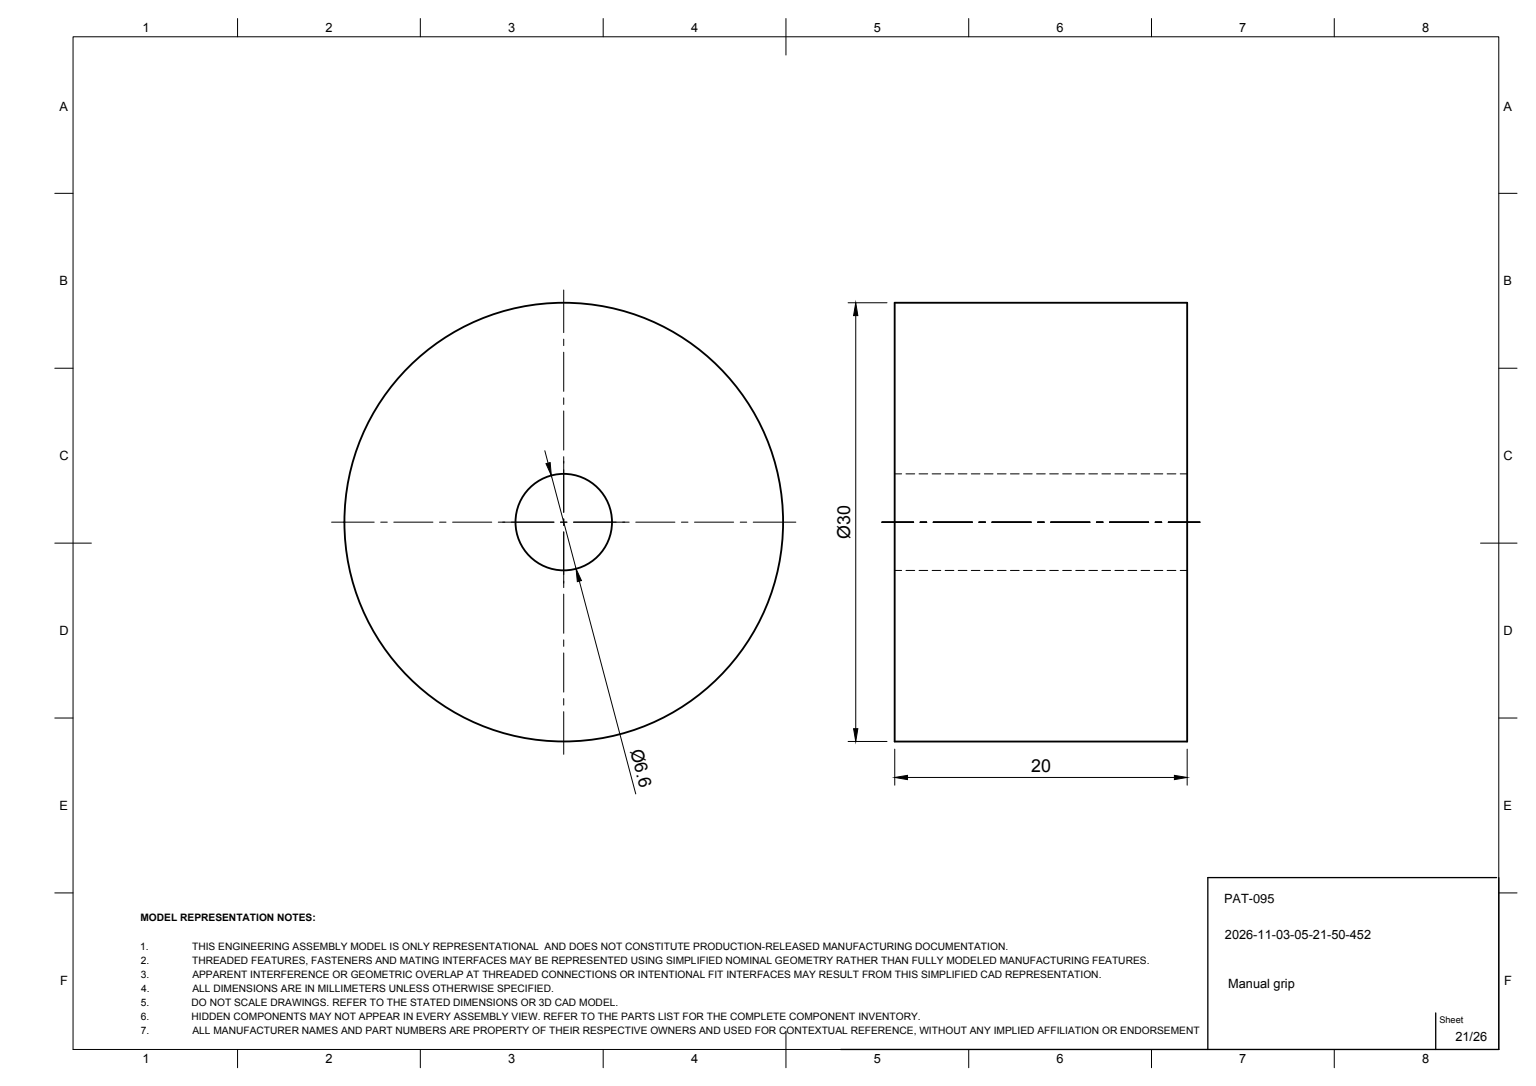
ISO-10303-21;
HEADER;
/* Generated by software containing ST-Developer
 * from STEP Tools, Inc. (www.steptools.com) 
 */

FILE_DESCRIPTION(
/* description */ ('Single-Axis Profile-Rail Linear Slide'),
/* implementation_level */ '2;1');

FILE_NAME(
/* name */ 'Manual grip.step',
/* time_stamp */ '2026-10-27T10:47:43-07:00',
/* author */ (''),
/* organization */ (''),
/* preprocessor_version */ 'ST-DEVELOPER v20.2',
/* originating_system */ 'Autodesk Translation Framework v15.17.0.0',
/* authorisation */ '');

FILE_SCHEMA (('AUTOMOTIVE_DESIGN { 1 0 10303 214 3 1 1 }'));
ENDSEC;

DATA;
#10=MECHANICAL_DESIGN_GEOMETRIC_PRESENTATION_REPRESENTATION('',(#346),#14478);
#292=SHAPE_REPRESENTATION_RELATIONSHIP('SRR','None',#14623,#319);
#319=ADVANCED_BREP_SHAPE_REPRESENTATION('',(#371),#14467);
#346=STYLED_ITEM('',(#14838),#371);
#371=MANIFOLD_SOLID_BREP('Body1',#8608);
#453=FACE_BOUND('',#1717,.T.);
#454=FACE_BOUND('',#1719,.T.);
#761=PLANE('',#9390);
#762=PLANE('',#9391);
#1184=FACE_OUTER_BOUND('',#1714,.T.);
#1185=FACE_OUTER_BOUND('',#1715,.T.);
#1186=FACE_OUTER_BOUND('',#1716,.T.);
#1187=FACE_OUTER_BOUND('',#1718,.T.);
#1714=EDGE_LOOP('',(#7583,#7584,#7585,#7586));
#1715=EDGE_LOOP('',(#7587,#7588,#7589,#7590));
#1716=EDGE_LOOP('',(#7591));
#1717=EDGE_LOOP('',(#7592));
#1718=EDGE_LOOP('',(#7593));
#1719=EDGE_LOOP('',(#7594));
#2625=LINE('',#13838,#3596);
#2626=LINE('',#13844,#3597);
#3596=VECTOR('',#11340,0.33);
#3597=VECTOR('',#11347,1.5);
#3880=CIRCLE('',#9385,0.33);
#3881=CIRCLE('',#9386,0.33);
#3882=CIRCLE('',#9388,1.5);
#3883=CIRCLE('',#9389,1.5);
#4526=VERTEX_POINT('',#13835);
#4527=VERTEX_POINT('',#13837);
#4528=VERTEX_POINT('',#13841);
#4529=VERTEX_POINT('',#13843);
#5569=EDGE_CURVE('',#4526,#4526,#3880,.T.);
#5570=EDGE_CURVE('',#4526,#4527,#2625,.T.);
#5571=EDGE_CURVE('',#4527,#4527,#3881,.T.);
#5572=EDGE_CURVE('',#4528,#4528,#3882,.T.);
#5573=EDGE_CURVE('',#4528,#4529,#2626,.T.);
#5574=EDGE_CURVE('',#4529,#4529,#3883,.T.);
#7583=ORIENTED_EDGE('',*,*,#5569,.F.);
#7584=ORIENTED_EDGE('',*,*,#5570,.T.);
#7585=ORIENTED_EDGE('',*,*,#5571,.T.);
#7586=ORIENTED_EDGE('',*,*,#5570,.F.);
#7587=ORIENTED_EDGE('',*,*,#5572,.F.);
#7588=ORIENTED_EDGE('',*,*,#5573,.T.);
#7589=ORIENTED_EDGE('',*,*,#5574,.T.);
#7590=ORIENTED_EDGE('',*,*,#5573,.F.);
#7591=ORIENTED_EDGE('',*,*,#5572,.T.);
#7592=ORIENTED_EDGE('',*,*,#5569,.T.);
#7593=ORIENTED_EDGE('',*,*,#5574,.F.);
#7594=ORIENTED_EDGE('',*,*,#5571,.F.);
#8116=CYLINDRICAL_SURFACE('',#9384,0.33);
#8117=CYLINDRICAL_SURFACE('',#9387,1.5);
#8478=ADVANCED_FACE('',(#1184),#8116,.F.);
#8479=ADVANCED_FACE('',(#1185),#8117,.T.);
#8480=ADVANCED_FACE('',(#1186,#453),#761,.T.);
#8481=ADVANCED_FACE('',(#1187,#454),#762,.F.);
#8608=CLOSED_SHELL('',(#8478,#8479,#8480,#8481));
#9383=AXIS2_PLACEMENT_3D('',#13833,#11334,#11335);
#9384=AXIS2_PLACEMENT_3D('',#13834,#11336,#11337);
#9385=AXIS2_PLACEMENT_3D('',#13836,#11338,#11339);
#9386=AXIS2_PLACEMENT_3D('',#13839,#11341,#11342);
#9387=AXIS2_PLACEMENT_3D('',#13840,#11343,#11344);
#9388=AXIS2_PLACEMENT_3D('',#13842,#11345,#11346);
#9389=AXIS2_PLACEMENT_3D('',#13845,#11348,#11349);
#9390=AXIS2_PLACEMENT_3D('',#13846,#11350,#11351);
#9391=AXIS2_PLACEMENT_3D('',#13847,#11352,#11353);
#11334=DIRECTION('axis',(0.,0.,1.));
#11335=DIRECTION('refdir',(1.,0.,0.));
#11336=DIRECTION('center_axis',(0.,0.,1.));
#11337=DIRECTION('ref_axis',(1.,0.,0.));
#11338=DIRECTION('center_axis',(0.,0.,-1.));
#11339=DIRECTION('ref_axis',(1.,0.,0.));
#11340=DIRECTION('',(0.,0.,-1.));
#11341=DIRECTION('center_axis',(0.,0.,-1.));
#11342=DIRECTION('ref_axis',(1.,0.,0.));
#11343=DIRECTION('center_axis',(0.,0.,1.));
#11344=DIRECTION('ref_axis',(1.,0.,0.));
#11345=DIRECTION('center_axis',(0.,0.,1.));
#11346=DIRECTION('ref_axis',(1.,0.,0.));
#11347=DIRECTION('',(0.,0.,-1.));
#11348=DIRECTION('center_axis',(0.,0.,1.));
#11349=DIRECTION('ref_axis',(1.,0.,0.));
#11350=DIRECTION('center_axis',(0.,0.,1.));
#11351=DIRECTION('ref_axis',(1.,0.,0.));
#11352=DIRECTION('center_axis',(0.,0.,1.));
#11353=DIRECTION('ref_axis',(1.,0.,0.));
#13833=CARTESIAN_POINT('',(0.,0.,0.));
#13834=CARTESIAN_POINT('Origin',(11.,0.,6.4));
#13835=CARTESIAN_POINT('',(10.67,-4.04133443718627E-17,8.4));
#13836=CARTESIAN_POINT('Origin',(11.,0.,8.4));
#13837=CARTESIAN_POINT('',(10.67,-4.04133443718627E-17,6.4));
#13838=CARTESIAN_POINT('',(10.67,-4.04133443718627E-17,6.4));
#13839=CARTESIAN_POINT('Origin',(11.,0.,6.4));
#13840=CARTESIAN_POINT('Origin',(11.,0.,6.4));
#13841=CARTESIAN_POINT('',(9.5,-1.83697019872103E-16,8.4));
#13842=CARTESIAN_POINT('Origin',(11.,0.,8.4));
#13843=CARTESIAN_POINT('',(9.5,-1.83697019872103E-16,6.4));
#13844=CARTESIAN_POINT('',(9.5,-1.83697019872103E-16,6.4));
#13845=CARTESIAN_POINT('Origin',(11.,0.,6.4));
#13846=CARTESIAN_POINT('Origin',(11.,0.,8.4));
#13847=CARTESIAN_POINT('Origin',(11.,0.,6.4));
#14435=UNCERTAINTY_MEASURE_WITH_UNIT(LENGTH_MEASURE(0.001),#14479,
'DISTANCE_ACCURACY_VALUE',
'Maximum model space distance between geometric entities at asserted c
onnectivities');
#14446=UNCERTAINTY_MEASURE_WITH_UNIT(LENGTH_MEASURE(0.001),#14479,
'DISTANCE_ACCURACY_VALUE',
'Maximum model space distance between geometric entities at asserted c
onnectivities');
#14467=(
GEOMETRIC_REPRESENTATION_CONTEXT(3)
GLOBAL_UNCERTAINTY_ASSIGNED_CONTEXT((#14435))
GLOBAL_UNIT_ASSIGNED_CONTEXT((#14479,#14481,#14482))
REPRESENTATION_CONTEXT('','3D')
);
#14478=(
GEOMETRIC_REPRESENTATION_CONTEXT(3)
GLOBAL_UNCERTAINTY_ASSIGNED_CONTEXT((#14446))
GLOBAL_UNIT_ASSIGNED_CONTEXT((#14479,#14481,#14482))
REPRESENTATION_CONTEXT('','3D')
);
#14479=(
LENGTH_UNIT()
NAMED_UNIT(*)
SI_UNIT(.CENTI.,.METRE.)
);
#14481=(
NAMED_UNIT(*)
PLANE_ANGLE_UNIT()
SI_UNIT($,.RADIAN.)
);
#14482=(
NAMED_UNIT(*)
SI_UNIT($,.STERADIAN.)
SOLID_ANGLE_UNIT()
);
#14503=SHAPE_DEFINITION_REPRESENTATION(#14534,#14623);
#14534=PRODUCT_DEFINITION_SHAPE('',$,#14655);
#14623=SHAPE_REPRESENTATION('',(#9383),#14467);
#14634=PRODUCT_DEFINITION_CONTEXT('part definition',#14729,'design');
#14655=PRODUCT_DEFINITION('Manual grip','Manual grip',#14686,#14634);
#14686=PRODUCT_DEFINITION_FORMATION('',$,#14751);
#14729=APPLICATION_CONTEXT(
'Core Data for Automotive Mechanical Design Process');
#14730=PRODUCT_CONTEXT('part definition',#14729,'mechanical');
#14751=PRODUCT('Manual grip','Manual grip','Manual grip',(#14730));
#14832=COLOUR_RGB('Black',0.12,0.14,0.17);
#14833=FILL_AREA_STYLE_COLOUR('',#14832);
#14834=FILL_AREA_STYLE('',(#14833));
#14835=SURFACE_STYLE_FILL_AREA(#14834);
#14836=SURFACE_SIDE_STYLE('',(#14835));
#14837=SURFACE_STYLE_USAGE(.BOTH.,#14836);
#14838=PRESENTATION_STYLE_ASSIGNMENT((#14837));
ENDSEC;
END-ISO-10303-21;
